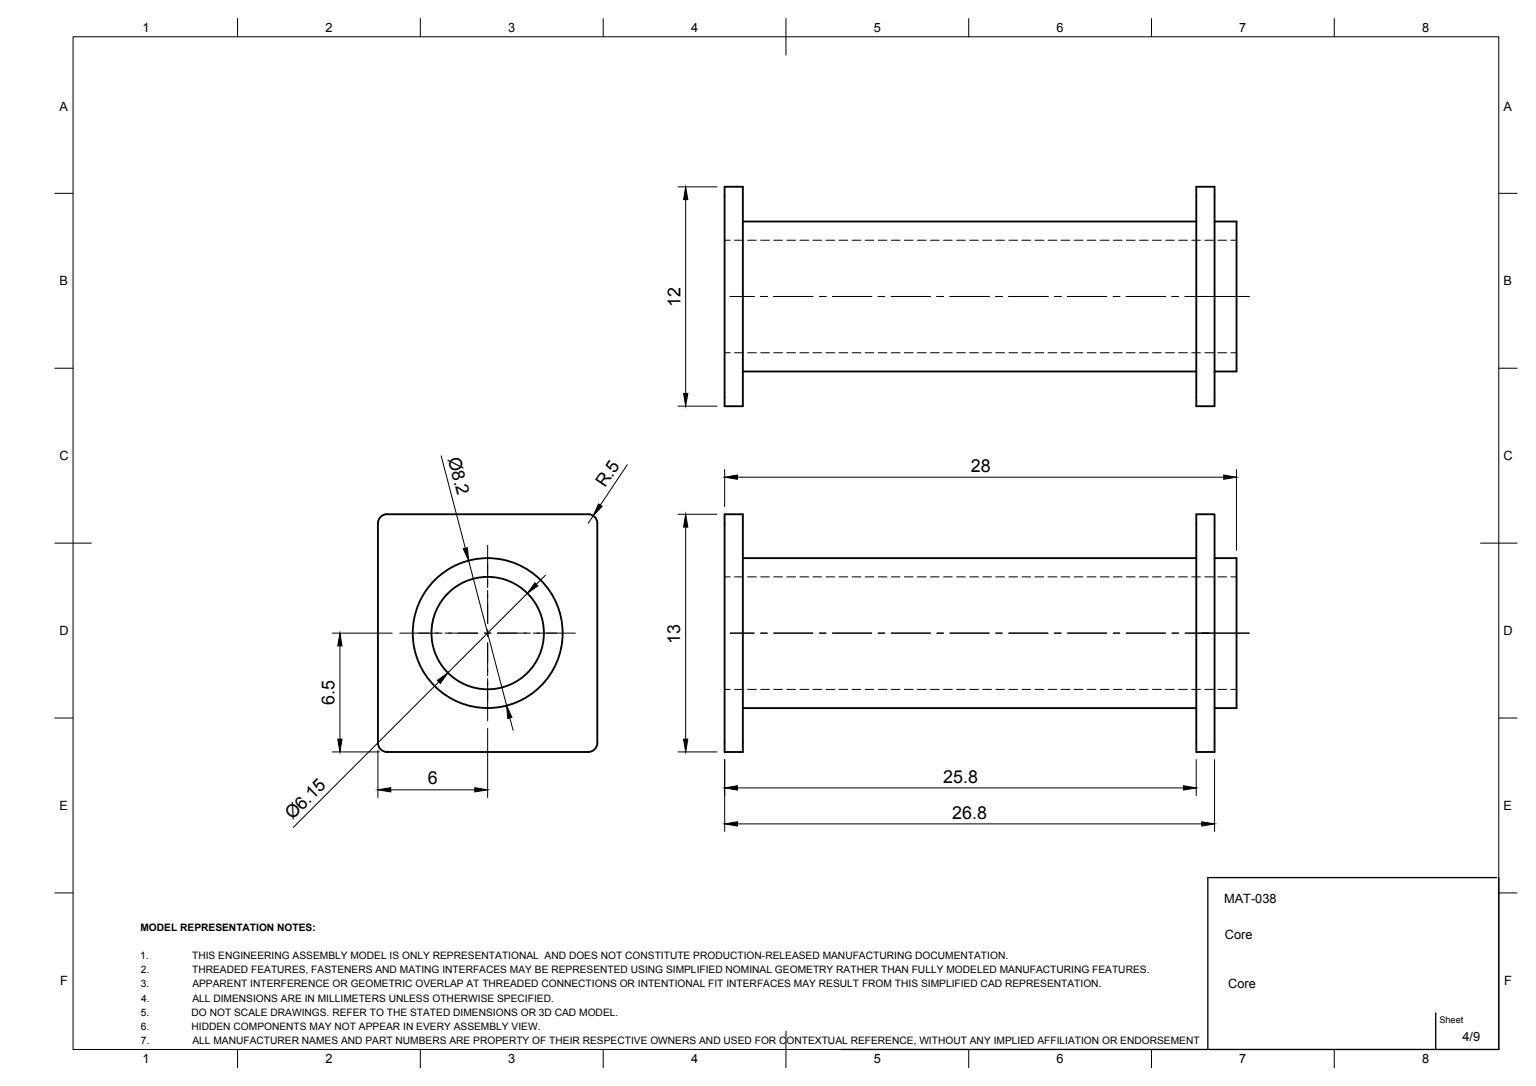
ISO-10303-21;
HEADER;
/* Generated by software containing ST-Developer
 * from STEP Tools, Inc. (www.steptools.com) 
 */

FILE_DESCRIPTION(
/* description */ ('STEP AP214'),
/* implementation_level */ '2;1');

FILE_NAME(
/* name */ 'Core.step',
/* time_stamp */ '2026-11-14T21:32:33-08:00',
/* author */ (''),
/* organization */ (''),
/* preprocessor_version */ 'ST-DEVELOPER v20.2',
/* originating_system */ 'Autodesk Translation Framework v15.17.0.0',
/* authorisation */ '');

FILE_SCHEMA (('AUTOMOTIVE_DESIGN { 1 0 10303 214 3 1 1 }'));
ENDSEC;

DATA;
#10=MECHANICAL_DESIGN_GEOMETRIC_PRESENTATION_REPRESENTATION('',(#178),#10551);
#160=SHAPE_REPRESENTATION_RELATIONSHIP('SRR','None',#10587,#169);
#169=ADVANCED_BREP_SHAPE_REPRESENTATION('',(#188),#10543);
#178=STYLED_ITEM('',(#10641),#188);
#188=MANIFOLD_SOLID_BREP('Body1',#3427);
#203=FACE_BOUND('',#549,.T.);
#204=FACE_BOUND('',#555,.T.);
#205=FACE_BOUND('',#557,.T.);
#206=FACE_BOUND('',#563,.T.);
#207=FACE_BOUND('',#565,.T.);
#242=PLANE('',#3587);
#243=PLANE('',#3588);
#244=PLANE('',#3589);
#245=PLANE('',#3590);
#246=PLANE('',#3591);
#247=PLANE('',#3592);
#248=PLANE('',#3597);
#249=PLANE('',#3602);
#250=PLANE('',#3603);
#251=PLANE('',#3604);
#252=PLANE('',#3605);
#253=PLANE('',#3606);
#254=PLANE('',#3611);
#319=FACE_OUTER_BOUND('',#545,.T.);
#320=FACE_OUTER_BOUND('',#546,.T.);
#321=FACE_OUTER_BOUND('',#547,.T.);
#322=FACE_OUTER_BOUND('',#548,.T.);
#323=FACE_OUTER_BOUND('',#550,.T.);
#324=FACE_OUTER_BOUND('',#551,.T.);
#325=FACE_OUTER_BOUND('',#552,.T.);
#326=FACE_OUTER_BOUND('',#553,.T.);
#327=FACE_OUTER_BOUND('',#554,.T.);
#328=FACE_OUTER_BOUND('',#556,.T.);
#329=FACE_OUTER_BOUND('',#558,.T.);
#330=FACE_OUTER_BOUND('',#559,.T.);
#331=FACE_OUTER_BOUND('',#560,.T.);
#332=FACE_OUTER_BOUND('',#561,.T.);
#333=FACE_OUTER_BOUND('',#562,.T.);
#334=FACE_OUTER_BOUND('',#564,.T.);
#335=FACE_OUTER_BOUND('',#566,.T.);
#336=FACE_OUTER_BOUND('',#567,.T.);
#337=FACE_OUTER_BOUND('',#568,.T.);
#338=FACE_OUTER_BOUND('',#569,.T.);
#339=FACE_OUTER_BOUND('',#570,.T.);
#340=FACE_OUTER_BOUND('',#571,.T.);
#341=FACE_OUTER_BOUND('',#572,.T.);
#342=FACE_OUTER_BOUND('',#573,.T.);
#545=EDGE_LOOP('',(#2326,#2327,#2328,#2329));
#546=EDGE_LOOP('',(#2330,#2331,#2332,#2333));
#547=EDGE_LOOP('',(#2334,#2335,#2336,#2337));
#548=EDGE_LOOP('',(#2338));
#549=EDGE_LOOP('',(#2339));
#550=EDGE_LOOP('',(#2340,#2341,#2342,#2343));
#551=EDGE_LOOP('',(#2344,#2345,#2346,#2347));
#552=EDGE_LOOP('',(#2348,#2349,#2350,#2351));
#553=EDGE_LOOP('',(#2352,#2353,#2354,#2355));
#554=EDGE_LOOP('',(#2356,#2357,#2358,#2359,#2360,#2361,#2362,#2363));
#555=EDGE_LOOP('',(#2364));
#556=EDGE_LOOP('',(#2365,#2366,#2367,#2368,#2369,#2370,#2371,#2372));
#557=EDGE_LOOP('',(#2373));
#558=EDGE_LOOP('',(#2374,#2375,#2376,#2377));
#559=EDGE_LOOP('',(#2378,#2379,#2380,#2381));
#560=EDGE_LOOP('',(#2382,#2383,#2384,#2385));
#561=EDGE_LOOP('',(#2386,#2387,#2388,#2389));
#562=EDGE_LOOP('',(#2390,#2391,#2392,#2393,#2394,#2395,#2396,#2397));
#563=EDGE_LOOP('',(#2398));
#564=EDGE_LOOP('',(#2399,#2400,#2401,#2402,#2403,#2404,#2405,#2406));
#565=EDGE_LOOP('',(#2407));
#566=EDGE_LOOP('',(#2408,#2409,#2410,#2411));
#567=EDGE_LOOP('',(#2412,#2413,#2414,#2415));
#568=EDGE_LOOP('',(#2416,#2417,#2418,#2419));
#569=EDGE_LOOP('',(#2420,#2421,#2422,#2423));
#570=EDGE_LOOP('',(#2424,#2425,#2426,#2427));
#571=EDGE_LOOP('',(#2428,#2429,#2430,#2431));
#572=EDGE_LOOP('',(#2432,#2433,#2434,#2435));
#573=EDGE_LOOP('',(#2436,#2437,#2438,#2439));
#816=LINE('',#5380,#1013);
#817=LINE('',#5386,#1014);
#818=LINE('',#5392,#1015);
#819=LINE('',#5398,#1016);
#820=LINE('',#5400,#1017);
#821=LINE('',#5402,#1018);
#822=LINE('',#5403,#1019);
#823=LINE('',#5407,#1020);
#824=LINE('',#5409,#1021);
#825=LINE('',#5411,#1022);
#826=LINE('',#5412,#1023);
#827=LINE('',#5416,#1024);
#828=LINE('',#5418,#1025);
#829=LINE('',#5420,#1026);
#830=LINE('',#5421,#1027);
#831=LINE('',#5425,#1028);
#832=LINE('',#5427,#1029);
#833=LINE('',#5429,#1030);
#834=LINE('',#5430,#1031);
#835=LINE('',#5444,#1032);
#836=LINE('',#5446,#1033);
#837=LINE('',#5448,#1034);
#838=LINE('',#5449,#1035);
#839=LINE('',#5453,#1036);
#840=LINE('',#5455,#1037);
#841=LINE('',#5457,#1038);
#842=LINE('',#5458,#1039);
#843=LINE('',#5462,#1040);
#844=LINE('',#5464,#1041);
#845=LINE('',#5466,#1042);
#846=LINE('',#5467,#1043);
#847=LINE('',#5471,#1044);
#848=LINE('',#5473,#1045);
#849=LINE('',#5475,#1046);
#850=LINE('',#5476,#1047);
#1013=VECTOR('',#4179,3.075);
#1014=VECTOR('',#4186,4.1);
#1015=VECTOR('',#4193,4.1);
#1016=VECTOR('',#4200,1000.);
#1017=VECTOR('',#4201,1000.);
#1018=VECTOR('',#4202,1000.);
#1019=VECTOR('',#4203,1000.);
#1020=VECTOR('',#4206,1000.);
#1021=VECTOR('',#4207,1000.);
#1022=VECTOR('',#4208,1000.);
#1023=VECTOR('',#4209,1000.);
#1024=VECTOR('',#4212,1000.);
#1025=VECTOR('',#4213,1000.);
#1026=VECTOR('',#4214,1000.);
#1027=VECTOR('',#4215,1000.);
#1028=VECTOR('',#4218,1000.);
#1029=VECTOR('',#4219,1000.);
#1030=VECTOR('',#4220,1000.);
#1031=VECTOR('',#4221,1000.);
#1032=VECTOR('',#4244,1000.);
#1033=VECTOR('',#4245,1000.);
#1034=VECTOR('',#4246,1000.);
#1035=VECTOR('',#4247,1000.);
#1036=VECTOR('',#4250,1000.);
#1037=VECTOR('',#4251,1000.);
#1038=VECTOR('',#4252,1000.);
#1039=VECTOR('',#4253,1000.);
#1040=VECTOR('',#4256,1000.);
#1041=VECTOR('',#4257,1000.);
#1042=VECTOR('',#4258,1000.);
#1043=VECTOR('',#4259,1000.);
#1044=VECTOR('',#4262,1000.);
#1045=VECTOR('',#4263,1000.);
#1046=VECTOR('',#4264,1000.);
#1047=VECTOR('',#4265,1000.);
#1169=CIRCLE('',#3579,3.075);
#1170=CIRCLE('',#3580,3.075);
#1171=CIRCLE('',#3582,4.1);
#1172=CIRCLE('',#3583,4.1);
#1173=CIRCLE('',#3585,4.1);
#1174=CIRCLE('',#3586,4.1);
#1175=CIRCLE('',#3593,0.5);
#1176=CIRCLE('',#3594,0.5);
#1177=CIRCLE('',#3595,0.5);
#1178=CIRCLE('',#3596,0.5);
#1179=CIRCLE('',#3598,0.5);
#1180=CIRCLE('',#3599,0.5);
#1181=CIRCLE('',#3600,0.5);
#1182=CIRCLE('',#3601,0.5);
#1183=CIRCLE('',#3607,0.5);
#1184=CIRCLE('',#3608,0.5);
#1185=CIRCLE('',#3609,0.5);
#1186=CIRCLE('',#3610,0.5);
#1187=CIRCLE('',#3612,0.5);
#1188=CIRCLE('',#3613,0.5);
#1189=CIRCLE('',#3614,0.5);
#1190=CIRCLE('',#3615,0.5);
#1467=VERTEX_POINT('',#5377);
#1468=VERTEX_POINT('',#5379);
#1469=VERTEX_POINT('',#5383);
#1470=VERTEX_POINT('',#5385);
#1471=VERTEX_POINT('',#5389);
#1472=VERTEX_POINT('',#5391);
#1473=VERTEX_POINT('',#5396);
#1474=VERTEX_POINT('',#5397);
#1475=VERTEX_POINT('',#5399);
#1476=VERTEX_POINT('',#5401);
#1477=VERTEX_POINT('',#5405);
#1478=VERTEX_POINT('',#5406);
#1479=VERTEX_POINT('',#5408);
#1480=VERTEX_POINT('',#5410);
#1481=VERTEX_POINT('',#5414);
#1482=VERTEX_POINT('',#5415);
#1483=VERTEX_POINT('',#5417);
#1484=VERTEX_POINT('',#5419);
#1485=VERTEX_POINT('',#5423);
#1486=VERTEX_POINT('',#5424);
#1487=VERTEX_POINT('',#5426);
#1488=VERTEX_POINT('',#5428);
#1489=VERTEX_POINT('',#5442);
#1490=VERTEX_POINT('',#5443);
#1491=VERTEX_POINT('',#5445);
#1492=VERTEX_POINT('',#5447);
#1493=VERTEX_POINT('',#5451);
#1494=VERTEX_POINT('',#5452);
#1495=VERTEX_POINT('',#5454);
#1496=VERTEX_POINT('',#5456);
#1497=VERTEX_POINT('',#5460);
#1498=VERTEX_POINT('',#5461);
#1499=VERTEX_POINT('',#5463);
#1500=VERTEX_POINT('',#5465);
#1501=VERTEX_POINT('',#5469);
#1502=VERTEX_POINT('',#5470);
#1503=VERTEX_POINT('',#5472);
#1504=VERTEX_POINT('',#5474);
#1776=EDGE_CURVE('',#1467,#1467,#1169,.T.);
#1777=EDGE_CURVE('',#1467,#1468,#816,.T.);
#1778=EDGE_CURVE('',#1468,#1468,#1170,.T.);
#1779=EDGE_CURVE('',#1469,#1469,#1171,.T.);
#1780=EDGE_CURVE('',#1469,#1470,#817,.T.);
#1781=EDGE_CURVE('',#1470,#1470,#1172,.T.);
#1782=EDGE_CURVE('',#1471,#1471,#1173,.T.);
#1783=EDGE_CURVE('',#1471,#1472,#818,.T.);
#1784=EDGE_CURVE('',#1472,#1472,#1174,.T.);
#1785=EDGE_CURVE('',#1473,#1474,#819,.T.);
#1786=EDGE_CURVE('',#1474,#1475,#820,.T.);
#1787=EDGE_CURVE('',#1476,#1475,#821,.T.);
#1788=EDGE_CURVE('',#1476,#1473,#822,.T.);
#1789=EDGE_CURVE('',#1477,#1478,#823,.T.);
#1790=EDGE_CURVE('',#1478,#1479,#824,.T.);
#1791=EDGE_CURVE('',#1480,#1479,#825,.T.);
#1792=EDGE_CURVE('',#1480,#1477,#826,.T.);
#1793=EDGE_CURVE('',#1481,#1482,#827,.T.);
#1794=EDGE_CURVE('',#1481,#1483,#828,.T.);
#1795=EDGE_CURVE('',#1483,#1484,#829,.T.);
#1796=EDGE_CURVE('',#1484,#1482,#830,.T.);
#1797=EDGE_CURVE('',#1485,#1486,#831,.T.);
#1798=EDGE_CURVE('',#1485,#1487,#832,.T.);
#1799=EDGE_CURVE('',#1487,#1488,#833,.T.);
#1800=EDGE_CURVE('',#1488,#1486,#834,.T.);
#1801=EDGE_CURVE('',#1479,#1481,#1175,.T.);
#1802=EDGE_CURVE('',#1482,#1485,#1176,.T.);
#1803=EDGE_CURVE('',#1486,#1476,#1177,.T.);
#1804=EDGE_CURVE('',#1475,#1480,#1178,.T.);
#1805=EDGE_CURVE('',#1483,#1478,#1179,.T.);
#1806=EDGE_CURVE('',#1477,#1474,#1180,.T.);
#1807=EDGE_CURVE('',#1473,#1488,#1181,.T.);
#1808=EDGE_CURVE('',#1487,#1484,#1182,.T.);
#1809=EDGE_CURVE('',#1489,#1490,#835,.T.);
#1810=EDGE_CURVE('',#1490,#1491,#836,.T.);
#1811=EDGE_CURVE('',#1492,#1491,#837,.T.);
#1812=EDGE_CURVE('',#1492,#1489,#838,.T.);
#1813=EDGE_CURVE('',#1493,#1494,#839,.T.);
#1814=EDGE_CURVE('',#1494,#1495,#840,.T.);
#1815=EDGE_CURVE('',#1496,#1495,#841,.T.);
#1816=EDGE_CURVE('',#1496,#1493,#842,.T.);
#1817=EDGE_CURVE('',#1497,#1498,#843,.T.);
#1818=EDGE_CURVE('',#1497,#1499,#844,.T.);
#1819=EDGE_CURVE('',#1499,#1500,#845,.T.);
#1820=EDGE_CURVE('',#1500,#1498,#846,.T.);
#1821=EDGE_CURVE('',#1501,#1502,#847,.T.);
#1822=EDGE_CURVE('',#1501,#1503,#848,.T.);
#1823=EDGE_CURVE('',#1503,#1504,#849,.T.);
#1824=EDGE_CURVE('',#1504,#1502,#850,.T.);
#1825=EDGE_CURVE('',#1503,#1490,#1183,.T.);
#1826=EDGE_CURVE('',#1489,#1494,#1184,.T.);
#1827=EDGE_CURVE('',#1493,#1500,#1185,.T.);
#1828=EDGE_CURVE('',#1499,#1504,#1186,.T.);
#1829=EDGE_CURVE('',#1491,#1501,#1187,.T.);
#1830=EDGE_CURVE('',#1502,#1497,#1188,.T.);
#1831=EDGE_CURVE('',#1498,#1496,#1189,.T.);
#1832=EDGE_CURVE('',#1495,#1492,#1190,.T.);
#2326=ORIENTED_EDGE('',*,*,#1776,.T.);
#2327=ORIENTED_EDGE('',*,*,#1777,.T.);
#2328=ORIENTED_EDGE('',*,*,#1778,.T.);
#2329=ORIENTED_EDGE('',*,*,#1777,.F.);
#2330=ORIENTED_EDGE('',*,*,#1779,.T.);
#2331=ORIENTED_EDGE('',*,*,#1780,.T.);
#2332=ORIENTED_EDGE('',*,*,#1781,.F.);
#2333=ORIENTED_EDGE('',*,*,#1780,.F.);
#2334=ORIENTED_EDGE('',*,*,#1782,.T.);
#2335=ORIENTED_EDGE('',*,*,#1783,.T.);
#2336=ORIENTED_EDGE('',*,*,#1784,.T.);
#2337=ORIENTED_EDGE('',*,*,#1783,.F.);
#2338=ORIENTED_EDGE('',*,*,#1784,.F.);
#2339=ORIENTED_EDGE('',*,*,#1778,.F.);
#2340=ORIENTED_EDGE('',*,*,#1785,.T.);
#2341=ORIENTED_EDGE('',*,*,#1786,.T.);
#2342=ORIENTED_EDGE('',*,*,#1787,.F.);
#2343=ORIENTED_EDGE('',*,*,#1788,.T.);
#2344=ORIENTED_EDGE('',*,*,#1789,.T.);
#2345=ORIENTED_EDGE('',*,*,#1790,.T.);
#2346=ORIENTED_EDGE('',*,*,#1791,.F.);
#2347=ORIENTED_EDGE('',*,*,#1792,.T.);
#2348=ORIENTED_EDGE('',*,*,#1793,.F.);
#2349=ORIENTED_EDGE('',*,*,#1794,.T.);
#2350=ORIENTED_EDGE('',*,*,#1795,.T.);
#2351=ORIENTED_EDGE('',*,*,#1796,.T.);
#2352=ORIENTED_EDGE('',*,*,#1797,.F.);
#2353=ORIENTED_EDGE('',*,*,#1798,.T.);
#2354=ORIENTED_EDGE('',*,*,#1799,.T.);
#2355=ORIENTED_EDGE('',*,*,#1800,.T.);
#2356=ORIENTED_EDGE('',*,*,#1791,.T.);
#2357=ORIENTED_EDGE('',*,*,#1801,.T.);
#2358=ORIENTED_EDGE('',*,*,#1793,.T.);
#2359=ORIENTED_EDGE('',*,*,#1802,.T.);
#2360=ORIENTED_EDGE('',*,*,#1797,.T.);
#2361=ORIENTED_EDGE('',*,*,#1803,.T.);
#2362=ORIENTED_EDGE('',*,*,#1787,.T.);
#2363=ORIENTED_EDGE('',*,*,#1804,.T.);
#2364=ORIENTED_EDGE('',*,*,#1782,.F.);
#2365=ORIENTED_EDGE('',*,*,#1795,.F.);
#2366=ORIENTED_EDGE('',*,*,#1805,.T.);
#2367=ORIENTED_EDGE('',*,*,#1789,.F.);
#2368=ORIENTED_EDGE('',*,*,#1806,.T.);
#2369=ORIENTED_EDGE('',*,*,#1785,.F.);
#2370=ORIENTED_EDGE('',*,*,#1807,.T.);
#2371=ORIENTED_EDGE('',*,*,#1799,.F.);
#2372=ORIENTED_EDGE('',*,*,#1808,.T.);
#2373=ORIENTED_EDGE('',*,*,#1781,.T.);
#2374=ORIENTED_EDGE('',*,*,#1809,.T.);
#2375=ORIENTED_EDGE('',*,*,#1810,.T.);
#2376=ORIENTED_EDGE('',*,*,#1811,.F.);
#2377=ORIENTED_EDGE('',*,*,#1812,.T.);
#2378=ORIENTED_EDGE('',*,*,#1813,.T.);
#2379=ORIENTED_EDGE('',*,*,#1814,.T.);
#2380=ORIENTED_EDGE('',*,*,#1815,.F.);
#2381=ORIENTED_EDGE('',*,*,#1816,.T.);
#2382=ORIENTED_EDGE('',*,*,#1817,.F.);
#2383=ORIENTED_EDGE('',*,*,#1818,.T.);
#2384=ORIENTED_EDGE('',*,*,#1819,.T.);
#2385=ORIENTED_EDGE('',*,*,#1820,.T.);
#2386=ORIENTED_EDGE('',*,*,#1821,.F.);
#2387=ORIENTED_EDGE('',*,*,#1822,.T.);
#2388=ORIENTED_EDGE('',*,*,#1823,.T.);
#2389=ORIENTED_EDGE('',*,*,#1824,.T.);
#2390=ORIENTED_EDGE('',*,*,#1823,.F.);
#2391=ORIENTED_EDGE('',*,*,#1825,.T.);
#2392=ORIENTED_EDGE('',*,*,#1809,.F.);
#2393=ORIENTED_EDGE('',*,*,#1826,.T.);
#2394=ORIENTED_EDGE('',*,*,#1813,.F.);
#2395=ORIENTED_EDGE('',*,*,#1827,.T.);
#2396=ORIENTED_EDGE('',*,*,#1819,.F.);
#2397=ORIENTED_EDGE('',*,*,#1828,.T.);
#2398=ORIENTED_EDGE('',*,*,#1779,.F.);
#2399=ORIENTED_EDGE('',*,*,#1811,.T.);
#2400=ORIENTED_EDGE('',*,*,#1829,.T.);
#2401=ORIENTED_EDGE('',*,*,#1821,.T.);
#2402=ORIENTED_EDGE('',*,*,#1830,.T.);
#2403=ORIENTED_EDGE('',*,*,#1817,.T.);
#2404=ORIENTED_EDGE('',*,*,#1831,.T.);
#2405=ORIENTED_EDGE('',*,*,#1815,.T.);
#2406=ORIENTED_EDGE('',*,*,#1832,.T.);
#2407=ORIENTED_EDGE('',*,*,#1776,.F.);
#2408=ORIENTED_EDGE('',*,*,#1825,.F.);
#2409=ORIENTED_EDGE('',*,*,#1822,.F.);
#2410=ORIENTED_EDGE('',*,*,#1829,.F.);
#2411=ORIENTED_EDGE('',*,*,#1810,.F.);
#2412=ORIENTED_EDGE('',*,*,#1828,.F.);
#2413=ORIENTED_EDGE('',*,*,#1818,.F.);
#2414=ORIENTED_EDGE('',*,*,#1830,.F.);
#2415=ORIENTED_EDGE('',*,*,#1824,.F.);
#2416=ORIENTED_EDGE('',*,*,#1826,.F.);
#2417=ORIENTED_EDGE('',*,*,#1812,.F.);
#2418=ORIENTED_EDGE('',*,*,#1832,.F.);
#2419=ORIENTED_EDGE('',*,*,#1814,.F.);
#2420=ORIENTED_EDGE('',*,*,#1827,.F.);
#2421=ORIENTED_EDGE('',*,*,#1816,.F.);
#2422=ORIENTED_EDGE('',*,*,#1831,.F.);
#2423=ORIENTED_EDGE('',*,*,#1820,.F.);
#2424=ORIENTED_EDGE('',*,*,#1801,.F.);
#2425=ORIENTED_EDGE('',*,*,#1790,.F.);
#2426=ORIENTED_EDGE('',*,*,#1805,.F.);
#2427=ORIENTED_EDGE('',*,*,#1794,.F.);
#2428=ORIENTED_EDGE('',*,*,#1804,.F.);
#2429=ORIENTED_EDGE('',*,*,#1786,.F.);
#2430=ORIENTED_EDGE('',*,*,#1806,.F.);
#2431=ORIENTED_EDGE('',*,*,#1792,.F.);
#2432=ORIENTED_EDGE('',*,*,#1802,.F.);
#2433=ORIENTED_EDGE('',*,*,#1796,.F.);
#2434=ORIENTED_EDGE('',*,*,#1808,.F.);
#2435=ORIENTED_EDGE('',*,*,#1798,.F.);
#2436=ORIENTED_EDGE('',*,*,#1803,.F.);
#2437=ORIENTED_EDGE('',*,*,#1800,.F.);
#2438=ORIENTED_EDGE('',*,*,#1807,.F.);
#2439=ORIENTED_EDGE('',*,*,#1788,.F.);
#3157=CYLINDRICAL_SURFACE('',#3578,3.075);
#3158=CYLINDRICAL_SURFACE('',#3581,4.1);
#3159=CYLINDRICAL_SURFACE('',#3584,4.1);
#3160=CYLINDRICAL_SURFACE('',#3616,0.5);
#3161=CYLINDRICAL_SURFACE('',#3617,0.5);
#3162=CYLINDRICAL_SURFACE('',#3618,0.5);
#3163=CYLINDRICAL_SURFACE('',#3619,0.5);
#3164=CYLINDRICAL_SURFACE('',#3620,0.5);
#3165=CYLINDRICAL_SURFACE('',#3621,0.5);
#3166=CYLINDRICAL_SURFACE('',#3622,0.5);
#3167=CYLINDRICAL_SURFACE('',#3623,0.5);
#3231=ADVANCED_FACE('',(#319),#3157,.F.);
#3232=ADVANCED_FACE('',(#320),#3158,.T.);
#3233=ADVANCED_FACE('',(#321),#3159,.T.);
#3234=ADVANCED_FACE('',(#322,#203),#242,.F.);
#3235=ADVANCED_FACE('',(#323),#243,.F.);
#3236=ADVANCED_FACE('',(#324),#244,.F.);
#3237=ADVANCED_FACE('',(#325),#245,.F.);
#3238=ADVANCED_FACE('',(#326),#246,.F.);
#3239=ADVANCED_FACE('',(#327,#204),#247,.T.);
#3240=ADVANCED_FACE('',(#328,#205),#248,.F.);
#3241=ADVANCED_FACE('',(#329),#249,.T.);
#3242=ADVANCED_FACE('',(#330),#250,.T.);
#3243=ADVANCED_FACE('',(#331),#251,.T.);
#3244=ADVANCED_FACE('',(#332),#252,.T.);
#3245=ADVANCED_FACE('',(#333,#206),#253,.T.);
#3246=ADVANCED_FACE('',(#334,#207),#254,.F.);
#3247=ADVANCED_FACE('',(#335),#3160,.T.);
#3248=ADVANCED_FACE('',(#336),#3161,.T.);
#3249=ADVANCED_FACE('',(#337),#3162,.T.);
#3250=ADVANCED_FACE('',(#338),#3163,.T.);
#3251=ADVANCED_FACE('',(#339),#3164,.T.);
#3252=ADVANCED_FACE('',(#340),#3165,.T.);
#3253=ADVANCED_FACE('',(#341),#3166,.T.);
#3254=ADVANCED_FACE('',(#342),#3167,.T.);
#3427=CLOSED_SHELL('',(#3231,#3232,#3233,#3234,#3235,#3236,#3237,#3238,
#3239,#3240,#3241,#3242,#3243,#3244,#3245,#3246,#3247,#3248,#3249,#3250,
#3251,#3252,#3253,#3254));
#3577=AXIS2_PLACEMENT_3D('',#5375,#4173,#4174);
#3578=AXIS2_PLACEMENT_3D('',#5376,#4175,#4176);
#3579=AXIS2_PLACEMENT_3D('',#5378,#4177,#4178);
#3580=AXIS2_PLACEMENT_3D('',#5381,#4180,#4181);
#3581=AXIS2_PLACEMENT_3D('',#5382,#4182,#4183);
#3582=AXIS2_PLACEMENT_3D('',#5384,#4184,#4185);
#3583=AXIS2_PLACEMENT_3D('',#5387,#4187,#4188);
#3584=AXIS2_PLACEMENT_3D('',#5388,#4189,#4190);
#3585=AXIS2_PLACEMENT_3D('',#5390,#4191,#4192);
#3586=AXIS2_PLACEMENT_3D('',#5393,#4194,#4195);
#3587=AXIS2_PLACEMENT_3D('',#5394,#4196,#4197);
#3588=AXIS2_PLACEMENT_3D('',#5395,#4198,#4199);
#3589=AXIS2_PLACEMENT_3D('',#5404,#4204,#4205);
#3590=AXIS2_PLACEMENT_3D('',#5413,#4210,#4211);
#3591=AXIS2_PLACEMENT_3D('',#5422,#4216,#4217);
#3592=AXIS2_PLACEMENT_3D('',#5431,#4222,#4223);
#3593=AXIS2_PLACEMENT_3D('',#5432,#4224,#4225);
#3594=AXIS2_PLACEMENT_3D('',#5433,#4226,#4227);
#3595=AXIS2_PLACEMENT_3D('',#5434,#4228,#4229);
#3596=AXIS2_PLACEMENT_3D('',#5435,#4230,#4231);
#3597=AXIS2_PLACEMENT_3D('',#5436,#4232,#4233);
#3598=AXIS2_PLACEMENT_3D('',#5437,#4234,#4235);
#3599=AXIS2_PLACEMENT_3D('',#5438,#4236,#4237);
#3600=AXIS2_PLACEMENT_3D('',#5439,#4238,#4239);
#3601=AXIS2_PLACEMENT_3D('',#5440,#4240,#4241);
#3602=AXIS2_PLACEMENT_3D('',#5441,#4242,#4243);
#3603=AXIS2_PLACEMENT_3D('',#5450,#4248,#4249);
#3604=AXIS2_PLACEMENT_3D('',#5459,#4254,#4255);
#3605=AXIS2_PLACEMENT_3D('',#5468,#4260,#4261);
#3606=AXIS2_PLACEMENT_3D('',#5477,#4266,#4267);
#3607=AXIS2_PLACEMENT_3D('',#5478,#4268,#4269);
#3608=AXIS2_PLACEMENT_3D('',#5479,#4270,#4271);
#3609=AXIS2_PLACEMENT_3D('',#5480,#4272,#4273);
#3610=AXIS2_PLACEMENT_3D('',#5481,#4274,#4275);
#3611=AXIS2_PLACEMENT_3D('',#5482,#4276,#4277);
#3612=AXIS2_PLACEMENT_3D('',#5483,#4278,#4279);
#3613=AXIS2_PLACEMENT_3D('',#5484,#4280,#4281);
#3614=AXIS2_PLACEMENT_3D('',#5485,#4282,#4283);
#3615=AXIS2_PLACEMENT_3D('',#5486,#4284,#4285);
#3616=AXIS2_PLACEMENT_3D('',#5487,#4286,#4287);
#3617=AXIS2_PLACEMENT_3D('',#5488,#4288,#4289);
#3618=AXIS2_PLACEMENT_3D('',#5489,#4290,#4291);
#3619=AXIS2_PLACEMENT_3D('',#5490,#4292,#4293);
#3620=AXIS2_PLACEMENT_3D('',#5491,#4294,#4295);
#3621=AXIS2_PLACEMENT_3D('',#5492,#4296,#4297);
#3622=AXIS2_PLACEMENT_3D('',#5493,#4298,#4299);
#3623=AXIS2_PLACEMENT_3D('',#5494,#4300,#4301);
#4173=DIRECTION('axis',(0.,0.,1.));
#4174=DIRECTION('refdir',(1.,0.,0.));
#4175=DIRECTION('center_axis',(1.,1.85863229568944E-16,0.));
#4176=DIRECTION('ref_axis',(-1.85863229568944E-16,1.,0.));
#4177=DIRECTION('center_axis',(-1.,-1.85863229568944E-16,0.));
#4178=DIRECTION('ref_axis',(-1.85863229568944E-16,1.,0.));
#4179=DIRECTION('',(1.,1.85863229568944E-16,0.));
#4180=DIRECTION('center_axis',(1.,1.85863229568944E-16,0.));
#4181=DIRECTION('ref_axis',(-1.85863229568944E-16,1.,0.));
#4182=DIRECTION('center_axis',(-1.,-1.85863229568944E-16,0.));
#4183=DIRECTION('ref_axis',(1.85863229568944E-16,-1.,0.));
#4184=DIRECTION('center_axis',(1.,2.66880534765663E-16,0.));
#4185=DIRECTION('ref_axis',(-2.66880534765663E-16,1.,0.));
#4186=DIRECTION('',(1.,1.85863229568944E-16,0.));
#4187=DIRECTION('center_axis',(1.,2.66880534765663E-16,0.));
#4188=DIRECTION('ref_axis',(-2.66880534765663E-16,1.,0.));
#4189=DIRECTION('center_axis',(-1.,-1.85863229568944E-16,0.));
#4190=DIRECTION('ref_axis',(1.85863229568944E-16,-1.,0.));
#4191=DIRECTION('center_axis',(1.,2.66880534765663E-16,0.));
#4192=DIRECTION('ref_axis',(-2.66880534765663E-16,1.,0.));
#4193=DIRECTION('',(1.,1.85863229568944E-16,0.));
#4194=DIRECTION('center_axis',(-1.,-1.85863229568944E-16,0.));
#4195=DIRECTION('ref_axis',(1.85863229568944E-16,-1.,0.));
#4196=DIRECTION('center_axis',(-1.,-1.85863229568944E-16,0.));
#4197=DIRECTION('ref_axis',(1.85863229568944E-16,-1.,0.));
#4198=DIRECTION('center_axis',(-2.48016390503164E-32,1.33440267382831E-16,
-1.));
#4199=DIRECTION('ref_axis',(0.,1.,1.33440267382831E-16));
#4200=DIRECTION('',(2.66880534765663E-16,-1.,-1.33440267382831E-16));
#4201=DIRECTION('',(1.,1.85863229568944E-16,5.47382212626882E-48));
#4202=DIRECTION('',(2.66880534765663E-16,-1.,-1.33440267382831E-16));
#4203=DIRECTION('',(-1.,-1.85863229568944E-16,-5.47382212626882E-48));
#4204=DIRECTION('center_axis',(-1.85863229568944E-16,1.,0.));
#4205=DIRECTION('ref_axis',(-1.,-1.85863229568944E-16,0.));
#4206=DIRECTION('',(0.,0.,-1.));
#4207=DIRECTION('',(1.,1.85863229568944E-16,5.47382212626882E-48));
#4208=DIRECTION('',(0.,0.,-1.));
#4209=DIRECTION('',(-1.,-1.85863229568944E-16,-5.47382212626882E-48));
#4210=DIRECTION('center_axis',(2.48016390503164E-32,-1.33440267382831E-16,
1.));
#4211=DIRECTION('ref_axis',(0.,-1.,-1.33440267382831E-16));
#4212=DIRECTION('',(-2.66880534765663E-16,1.,1.33440267382831E-16));
#4213=DIRECTION('',(-1.,-1.85863229568944E-16,-5.47382212626882E-48));
#4214=DIRECTION('',(-2.66880534765663E-16,1.,1.33440267382831E-16));
#4215=DIRECTION('',(1.,1.85863229568944E-16,5.47382212626882E-48));
#4216=DIRECTION('center_axis',(1.85863229568944E-16,-1.,0.));
#4217=DIRECTION('ref_axis',(1.,1.85863229568944E-16,0.));
#4218=DIRECTION('',(0.,0.,1.));
#4219=DIRECTION('',(-1.,-1.85863229568944E-16,-5.47382212626882E-48));
#4220=DIRECTION('',(0.,0.,1.));
#4221=DIRECTION('',(1.,1.85863229568944E-16,5.47382212626882E-48));
#4222=DIRECTION('center_axis',(1.,2.66880534765663E-16,0.));
#4223=DIRECTION('ref_axis',(-2.66880534765663E-16,1.,0.));
#4224=DIRECTION('center_axis',(1.,2.66880534765663E-16,0.));
#4225=DIRECTION('ref_axis',(-2.66880534765663E-16,1.,0.));
#4226=DIRECTION('center_axis',(1.,2.66880534765663E-16,0.));
#4227=DIRECTION('ref_axis',(-2.66880534765663E-16,1.,0.));
#4228=DIRECTION('center_axis',(1.,2.66880534765663E-16,0.));
#4229=DIRECTION('ref_axis',(-2.66880534765663E-16,1.,0.));
#4230=DIRECTION('center_axis',(1.,2.66880534765663E-16,0.));
#4231=DIRECTION('ref_axis',(-2.66880534765663E-16,1.,0.));
#4232=DIRECTION('center_axis',(1.,2.66880534765663E-16,0.));
#4233=DIRECTION('ref_axis',(-2.66880534765663E-16,1.,0.));
#4234=DIRECTION('center_axis',(-1.,-2.66880534765663E-16,0.));
#4235=DIRECTION('ref_axis',(-2.66880534765663E-16,1.,0.));
#4236=DIRECTION('center_axis',(-1.,-2.66880534765663E-16,0.));
#4237=DIRECTION('ref_axis',(-2.66880534765663E-16,1.,0.));
#4238=DIRECTION('center_axis',(-1.,-2.66880534765663E-16,0.));
#4239=DIRECTION('ref_axis',(-2.66880534765663E-16,1.,0.));
#4240=DIRECTION('center_axis',(-1.,-2.66880534765663E-16,0.));
#4241=DIRECTION('ref_axis',(-2.66880534765663E-16,1.,0.));
#4242=DIRECTION('center_axis',(-2.48016390503164E-32,1.33440267382831E-16,
-1.));
#4243=DIRECTION('ref_axis',(0.,1.,1.33440267382831E-16));
#4244=DIRECTION('',(2.66880534765663E-16,-1.,-1.33440267382831E-16));
#4245=DIRECTION('',(-1.,-1.85863229568944E-16,-5.47382212626882E-48));
#4246=DIRECTION('',(2.66880534765663E-16,-1.,-1.33440267382831E-16));
#4247=DIRECTION('',(1.,1.85863229568944E-16,5.47382212626882E-48));
#4248=DIRECTION('center_axis',(-1.85863229568944E-16,1.,0.));
#4249=DIRECTION('ref_axis',(-1.,-1.85863229568944E-16,0.));
#4250=DIRECTION('',(0.,0.,-1.));
#4251=DIRECTION('',(-1.,-1.85863229568944E-16,-5.47382212626882E-48));
#4252=DIRECTION('',(0.,0.,-1.));
#4253=DIRECTION('',(1.,1.85863229568944E-16,5.47382212626882E-48));
#4254=DIRECTION('center_axis',(2.48016390503164E-32,-1.33440267382831E-16,
1.));
#4255=DIRECTION('ref_axis',(0.,-1.,-1.33440267382831E-16));
#4256=DIRECTION('',(-2.66880534765663E-16,1.,1.33440267382831E-16));
#4257=DIRECTION('',(1.,1.85863229568944E-16,5.47382212626882E-48));
#4258=DIRECTION('',(-2.66880534765663E-16,1.,1.33440267382831E-16));
#4259=DIRECTION('',(-1.,-1.85863229568944E-16,-5.47382212626882E-48));
#4260=DIRECTION('center_axis',(1.85863229568944E-16,-1.,0.));
#4261=DIRECTION('ref_axis',(1.,1.85863229568944E-16,0.));
#4262=DIRECTION('',(0.,0.,1.));
#4263=DIRECTION('',(1.,1.85863229568944E-16,5.47382212626882E-48));
#4264=DIRECTION('',(0.,0.,1.));
#4265=DIRECTION('',(-1.,-1.85863229568944E-16,-5.47382212626882E-48));
#4266=DIRECTION('center_axis',(1.,2.66880534765663E-16,0.));
#4267=DIRECTION('ref_axis',(-2.66880534765663E-16,1.,0.));
#4268=DIRECTION('center_axis',(1.,2.66880534765663E-16,0.));
#4269=DIRECTION('ref_axis',(-2.66880534765663E-16,1.,0.));
#4270=DIRECTION('center_axis',(1.,2.66880534765663E-16,0.));
#4271=DIRECTION('ref_axis',(-2.66880534765663E-16,1.,0.));
#4272=DIRECTION('center_axis',(1.,2.66880534765663E-16,0.));
#4273=DIRECTION('ref_axis',(-2.66880534765663E-16,1.,0.));
#4274=DIRECTION('center_axis',(1.,2.66880534765663E-16,0.));
#4275=DIRECTION('ref_axis',(-2.66880534765663E-16,1.,0.));
#4276=DIRECTION('center_axis',(1.,1.85863229568944E-16,0.));
#4277=DIRECTION('ref_axis',(-1.85863229568944E-16,1.,0.));
#4278=DIRECTION('center_axis',(-1.,-1.85863229568944E-16,0.));
#4279=DIRECTION('ref_axis',(-1.85863229568944E-16,1.,0.));
#4280=DIRECTION('center_axis',(-1.,-1.85863229568944E-16,0.));
#4281=DIRECTION('ref_axis',(-1.85863229568944E-16,1.,0.));
#4282=DIRECTION('center_axis',(-1.,-1.85863229568944E-16,0.));
#4283=DIRECTION('ref_axis',(-1.85863229568944E-16,1.,5.20417042793042E-15));
#4284=DIRECTION('center_axis',(-1.,-1.85863229568944E-16,0.));
#4285=DIRECTION('ref_axis',(-1.85863229568944E-16,1.,0.));
#4286=DIRECTION('center_axis',(-1.,-1.85863229568944E-16,-5.47382212626882E-48));
#4287=DIRECTION('ref_axis',(1.85863229568944E-16,-1.,1.01738225847426E-63));
#4288=DIRECTION('center_axis',(-1.,-1.85863229568944E-16,-5.47382212626882E-48));
#4289=DIRECTION('ref_axis',(1.85863229568944E-16,-1.,1.01738225847426E-63));
#4290=DIRECTION('center_axis',(-1.,-1.85863229568944E-16,-5.47382212626882E-48));
#4291=DIRECTION('ref_axis',(1.85863229568944E-16,-1.,1.01738225847426E-63));
#4292=DIRECTION('center_axis',(-1.,-1.85863229568944E-16,-5.47382212626882E-48));
#4293=DIRECTION('ref_axis',(1.85863229568944E-16,-1.,1.01738225847426E-63));
#4294=DIRECTION('center_axis',(-1.,-1.85863229568944E-16,-5.47382212626882E-48));
#4295=DIRECTION('ref_axis',(1.85863229568944E-16,-1.,1.01738225847426E-63));
#4296=DIRECTION('center_axis',(-1.,-1.85863229568944E-16,-5.47382212626882E-48));
#4297=DIRECTION('ref_axis',(1.85863229568944E-16,-1.,1.01738225847426E-63));
#4298=DIRECTION('center_axis',(-1.,-1.85863229568944E-16,-5.47382212626882E-48));
#4299=DIRECTION('ref_axis',(1.85863229568944E-16,-1.,1.01738225847426E-63));
#4300=DIRECTION('center_axis',(-1.,-1.85863229568944E-16,-5.47382212626882E-48));
#4301=DIRECTION('ref_axis',(1.85863229568944E-16,-1.,1.01738225847426E-63));
#5375=CARTESIAN_POINT('',(0.,0.,0.));
#5376=CARTESIAN_POINT('Origin',(-14.001,-1.85863229568951E-19,0.));
#5377=CARTESIAN_POINT('',(-14.,-3.075,-3.76578890737811E-16));
#5378=CARTESIAN_POINT('Origin',(-14.,5.01301320851673E-31,0.));
#5379=CARTESIAN_POINT('',(14.,-3.075,-3.76578890737811E-16));
#5380=CARTESIAN_POINT('',(-14.001,-3.075,-3.76578890737811E-16));
#5381=CARTESIAN_POINT('Origin',(14.,5.20417042793042E-15,0.));
#5382=CARTESIAN_POINT('Origin',(-14.,0.,0.));
#5383=CARTESIAN_POINT('',(-13.,4.1,-5.02105187650415E-16));
#5384=CARTESIAN_POINT('Origin',(-13.,1.85863229568944E-16,0.));
#5385=CARTESIAN_POINT('',(11.8,4.1,-5.02105187650415E-16));
#5386=CARTESIAN_POINT('',(-14.,4.1,-5.02105187650415E-16));
#5387=CARTESIAN_POINT('Origin',(11.8,4.79527132287875E-15,0.));
#5388=CARTESIAN_POINT('Origin',(-14.,0.,0.));
#5389=CARTESIAN_POINT('',(12.8,4.1,-5.02105187650415E-16));
#5390=CARTESIAN_POINT('Origin',(12.8,4.98113455244769E-15,0.));
#5391=CARTESIAN_POINT('',(14.,4.1,-5.02105187650415E-16));
#5392=CARTESIAN_POINT('',(-14.,4.1,-5.02105187650415E-16));
#5393=CARTESIAN_POINT('Origin',(14.,5.20417042793042E-15,0.));
#5394=CARTESIAN_POINT('Origin',(14.,5.20417042793042E-15,0.));
#5395=CARTESIAN_POINT('Origin',(12.8,6.5,6.));
#5396=CARTESIAN_POINT('',(11.8,6.,6.));
#5397=CARTESIAN_POINT('',(11.8,-5.99999999999999,6.));
#5398=CARTESIAN_POINT('',(11.8,6.5,6.));
#5399=CARTESIAN_POINT('',(12.8,-5.99999999999999,6.));
#5400=CARTESIAN_POINT('',(12.8,-6.,6.));
#5401=CARTESIAN_POINT('',(12.8,6.,6.));
#5402=CARTESIAN_POINT('',(12.8,6.5,6.));
#5403=CARTESIAN_POINT('',(12.8,6.,6.));
#5404=CARTESIAN_POINT('Origin',(12.8,-6.5,6.));
#5405=CARTESIAN_POINT('',(11.8,-6.5,5.5));
#5406=CARTESIAN_POINT('',(11.8,-6.5,-5.5));
#5407=CARTESIAN_POINT('',(11.8,-6.5,6.));
#5408=CARTESIAN_POINT('',(12.8,-6.5,-5.5));
#5409=CARTESIAN_POINT('',(12.8,-6.5,-5.5));
#5410=CARTESIAN_POINT('',(12.8,-6.5,5.5));
#5411=CARTESIAN_POINT('',(12.8,-6.5,6.));
#5412=CARTESIAN_POINT('',(12.8,-6.5,5.5));
#5413=CARTESIAN_POINT('Origin',(12.8,6.5,-6.));
#5414=CARTESIAN_POINT('',(12.8,-5.99999999999999,-6.));
#5415=CARTESIAN_POINT('',(12.8,6.,-6.));
#5416=CARTESIAN_POINT('',(12.8,6.5,-6.));
#5417=CARTESIAN_POINT('',(11.8,-5.99999999999999,-6.));
#5418=CARTESIAN_POINT('',(12.8,-6.,-6.));
#5419=CARTESIAN_POINT('',(11.8,6.,-6.));
#5420=CARTESIAN_POINT('',(11.8,6.5,-6.));
#5421=CARTESIAN_POINT('',(12.8,6.,-6.));
#5422=CARTESIAN_POINT('Origin',(12.8,6.5,6.));
#5423=CARTESIAN_POINT('',(12.8,6.5,-5.5));
#5424=CARTESIAN_POINT('',(12.8,6.5,5.5));
#5425=CARTESIAN_POINT('',(12.8,6.5,6.));
#5426=CARTESIAN_POINT('',(11.8,6.5,-5.5));
#5427=CARTESIAN_POINT('',(12.8,6.5,-5.5));
#5428=CARTESIAN_POINT('',(11.8,6.5,5.5));
#5429=CARTESIAN_POINT('',(11.8,6.5,6.));
#5430=CARTESIAN_POINT('',(12.8,6.5,5.5));
#5431=CARTESIAN_POINT('Origin',(12.8,3.33505353980376E-15,0.));
#5432=CARTESIAN_POINT('Origin',(12.8,-6.,-5.5));
#5433=CARTESIAN_POINT('Origin',(12.8,6.,-5.5));
#5434=CARTESIAN_POINT('Origin',(12.8,6.,5.5));
#5435=CARTESIAN_POINT('Origin',(12.8,-6.,5.5));
#5436=CARTESIAN_POINT('Origin',(11.8,3.14919031023482E-15,0.));
#5437=CARTESIAN_POINT('Origin',(11.8,-6.,-5.5));
#5438=CARTESIAN_POINT('Origin',(11.8,-6.,5.5));
#5439=CARTESIAN_POINT('Origin',(11.8,6.,5.5));
#5440=CARTESIAN_POINT('Origin',(11.8,6.,-5.5));
#5441=CARTESIAN_POINT('Origin',(-13.,-6.5,-6.));
#5442=CARTESIAN_POINT('',(-13.,5.99999999999999,-6.));
#5443=CARTESIAN_POINT('',(-13.,-6.,-6.));
#5444=CARTESIAN_POINT('',(-13.,-6.5,-6.));
#5445=CARTESIAN_POINT('',(-14.,-6.,-6.));
#5446=CARTESIAN_POINT('',(-13.,-6.,-6.));
#5447=CARTESIAN_POINT('',(-14.,5.99999999999999,-6.));
#5448=CARTESIAN_POINT('',(-14.,-6.5,-6.));
#5449=CARTESIAN_POINT('',(-13.,6.,-6.));
#5450=CARTESIAN_POINT('Origin',(-13.,6.5,-6.));
#5451=CARTESIAN_POINT('',(-13.,6.5,5.5));
#5452=CARTESIAN_POINT('',(-13.,6.5,-5.5));
#5453=CARTESIAN_POINT('',(-13.,6.5,-6.));
#5454=CARTESIAN_POINT('',(-14.,6.5,-5.5));
#5455=CARTESIAN_POINT('',(-13.,6.5,-5.5));
#5456=CARTESIAN_POINT('',(-14.,6.5,5.5));
#5457=CARTESIAN_POINT('',(-14.,6.5,-6.));
#5458=CARTESIAN_POINT('',(-13.,6.5,5.5));
#5459=CARTESIAN_POINT('Origin',(-13.,6.5,6.));
#5460=CARTESIAN_POINT('',(-14.,-6.,6.));
#5461=CARTESIAN_POINT('',(-14.,6.,6.));
#5462=CARTESIAN_POINT('',(-14.,6.5,6.));
#5463=CARTESIAN_POINT('',(-13.,-6.,6.));
#5464=CARTESIAN_POINT('',(-13.,-6.,6.));
#5465=CARTESIAN_POINT('',(-13.,6.,6.));
#5466=CARTESIAN_POINT('',(-13.,6.5,6.));
#5467=CARTESIAN_POINT('',(-13.,6.,6.));
#5468=CARTESIAN_POINT('Origin',(-13.,-6.5,6.));
#5469=CARTESIAN_POINT('',(-14.,-6.5,-5.5));
#5470=CARTESIAN_POINT('',(-14.,-6.5,5.5));
#5471=CARTESIAN_POINT('',(-14.,-6.5,6.));
#5472=CARTESIAN_POINT('',(-13.,-6.5,-5.5));
#5473=CARTESIAN_POINT('',(-13.,-6.5,-5.5));
#5474=CARTESIAN_POINT('',(-13.,-6.5,5.5));
#5475=CARTESIAN_POINT('',(-13.,-6.5,6.));
#5476=CARTESIAN_POINT('',(-13.,-6.5,5.5));
#5477=CARTESIAN_POINT('Origin',(-13.,-3.55046425715033E-15,0.));
#5478=CARTESIAN_POINT('Origin',(-13.,-6.,-5.5));
#5479=CARTESIAN_POINT('Origin',(-13.,6.,-5.5));
#5480=CARTESIAN_POINT('Origin',(-13.,6.,5.5));
#5481=CARTESIAN_POINT('Origin',(-13.,-6.,5.5));
#5482=CARTESIAN_POINT('Origin',(-14.,7.08175372168856E-32,0.));
#5483=CARTESIAN_POINT('Origin',(-14.,-6.,-5.5));
#5484=CARTESIAN_POINT('Origin',(-14.,-6.,5.5));
#5485=CARTESIAN_POINT('Origin',(-14.,6.,5.5));
#5486=CARTESIAN_POINT('Origin',(-14.,6.,-5.5));
#5487=CARTESIAN_POINT('Origin',(-13.,-6.,-5.5));
#5488=CARTESIAN_POINT('Origin',(-13.,-6.,5.5));
#5489=CARTESIAN_POINT('Origin',(-13.,6.,-5.5));
#5490=CARTESIAN_POINT('Origin',(-13.,6.,5.5));
#5491=CARTESIAN_POINT('Origin',(12.8,-6.,-5.5));
#5492=CARTESIAN_POINT('Origin',(12.8,-6.,5.5));
#5493=CARTESIAN_POINT('Origin',(12.8,6.,-5.5));
#5494=CARTESIAN_POINT('Origin',(12.8,6.,5.5));
#10532=UNCERTAINTY_MEASURE_WITH_UNIT(LENGTH_MEASURE(0.01),#10552,
'DISTANCE_ACCURACY_VALUE',
'Maximum model space distance between geometric entities at asserted c
onnectivities');
#10540=UNCERTAINTY_MEASURE_WITH_UNIT(LENGTH_MEASURE(0.01),#10552,
'DISTANCE_ACCURACY_VALUE',
'Maximum model space distance between geometric entities at asserted c
onnectivities');
#10543=(
GEOMETRIC_REPRESENTATION_CONTEXT(3)
GLOBAL_UNCERTAINTY_ASSIGNED_CONTEXT((#10532))
GLOBAL_UNIT_ASSIGNED_CONTEXT((#10552,#10554,#10555))
REPRESENTATION_CONTEXT('','3D')
);
#10551=(
GEOMETRIC_REPRESENTATION_CONTEXT(3)
GLOBAL_UNCERTAINTY_ASSIGNED_CONTEXT((#10540))
GLOBAL_UNIT_ASSIGNED_CONTEXT((#10552,#10554,#10555))
REPRESENTATION_CONTEXT('','3D')
);
#10552=(
LENGTH_UNIT()
NAMED_UNIT(*)
SI_UNIT(.MILLI.,.METRE.)
);
#10554=(
NAMED_UNIT(*)
PLANE_ANGLE_UNIT()
SI_UNIT($,.RADIAN.)
);
#10555=(
NAMED_UNIT(*)
SI_UNIT($,.STERADIAN.)
SOLID_ANGLE_UNIT()
);
#10558=SHAPE_DEFINITION_REPRESENTATION(#10568,#10587);
#10568=PRODUCT_DEFINITION_SHAPE('',$,#10598);
#10587=SHAPE_REPRESENTATION('',(#3577),#10543);
#10595=PRODUCT_DEFINITION_CONTEXT('part definition',#10627,'design');
#10598=PRODUCT_DEFINITION('Core','Core',#10608,#10595);
#10608=PRODUCT_DEFINITION_FORMATION('',$,#10631);
#10627=APPLICATION_CONTEXT(
'Core Data for Automotive Mechanical Design Process');
#10628=PRODUCT_CONTEXT('part definition',#10627,'mechanical');
#10631=PRODUCT('Core','Core',$,(#10628));
#10641=PRESENTATION_STYLE_ASSIGNMENT((#10648));
#10648=SURFACE_STYLE_USAGE(.BOTH.,#10655);
#10655=SURFACE_SIDE_STYLE('',(#10662));
#10662=SURFACE_STYLE_FILL_AREA(#10669);
#10669=FILL_AREA_STYLE('Opaque(97,158,199)',(#10676));
#10676=FILL_AREA_STYLE_COLOUR('Opaque(97,158,199)',#10683);
#10683=COLOUR_RGB('Opaque(97,158,199)',0.380392156862745,0.619607843137255,
0.780392156862745);
ENDSEC;
END-ISO-10303-21;
